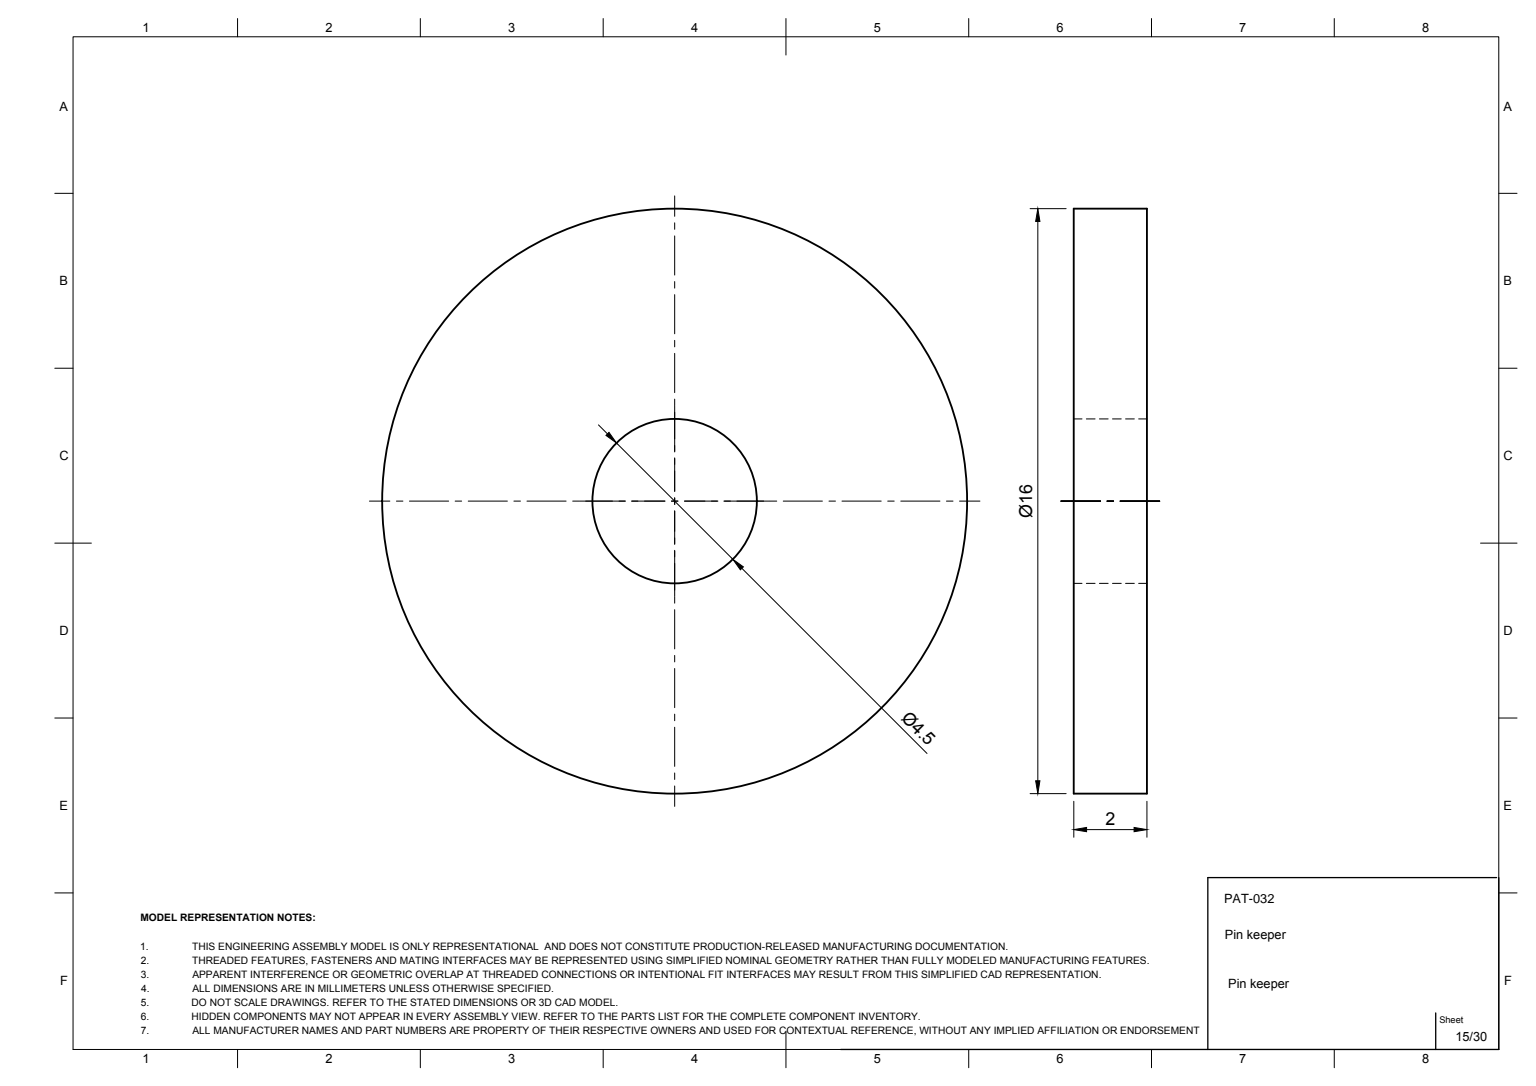
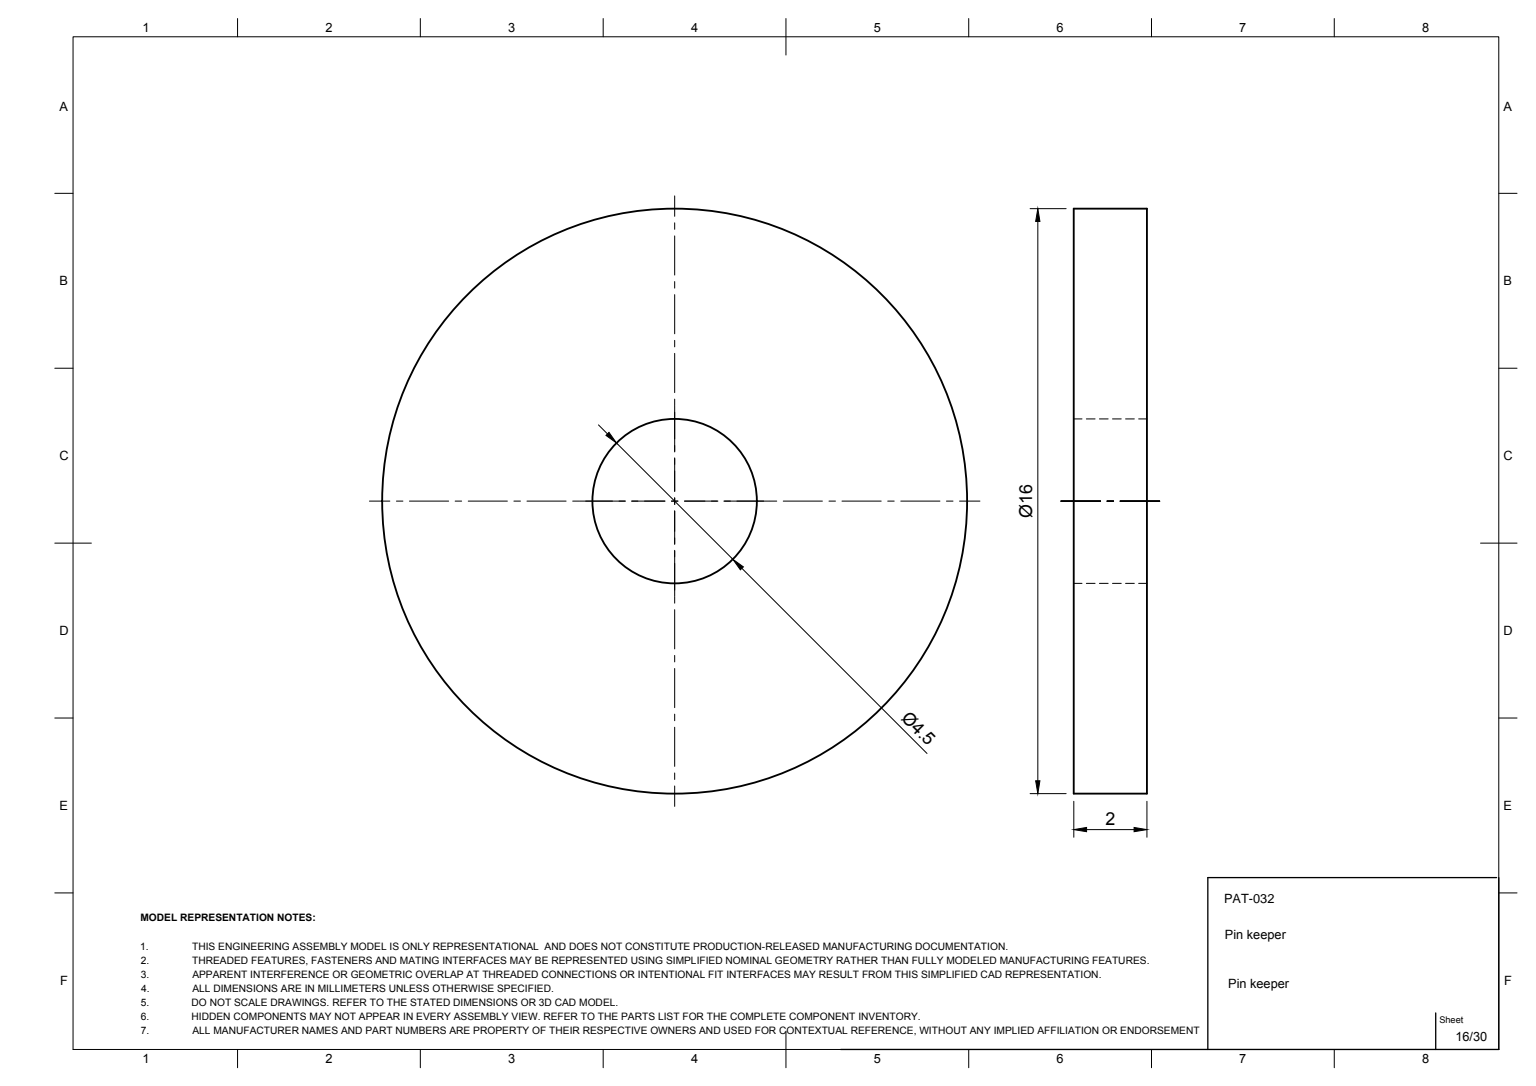
ISO-10303-21;
HEADER;
/* Generated by software containing ST-Developer
 * from STEP Tools, Inc. (www.steptools.com) 
 */

FILE_DESCRIPTION(
/* description */ ('Drill jig with bushing plate'),
/* implementation_level */ '2;1');

FILE_NAME(
/* name */ 'Pin keeper.step',
/* time_stamp */ '2026-10-27T10:51:08-07:00',
/* author */ (''),
/* organization */ (''),
/* preprocessor_version */ 'ST-DEVELOPER v20.2',
/* originating_system */ 'Autodesk Translation Framework v15.17.0.0',
/* authorisation */ '');

FILE_SCHEMA (('AUTOMOTIVE_DESIGN { 1 0 10303 214 3 1 1 }'));
ENDSEC;

DATA;
#10=MECHANICAL_DESIGN_GEOMETRIC_PRESENTATION_REPRESENTATION('',(#233),#6638);
#185=SHAPE_REPRESENTATION_RELATIONSHIP('SRR','None',#6749,#209);
#209=ADVANCED_BREP_SHAPE_REPRESENTATION('',(#257),#6622);
#233=STYLED_ITEM('',(#6943),#257);
#257=MANIFOLD_SOLID_BREP('Body1',#3600);
#330=FACE_BOUND('',#873,.T.);
#331=FACE_BOUND('',#875,.T.);
#427=PLANE('',#4068);
#428=PLANE('',#4069);
#595=FACE_OUTER_BOUND('',#870,.T.);
#596=FACE_OUTER_BOUND('',#871,.T.);
#597=FACE_OUTER_BOUND('',#872,.T.);
#598=FACE_OUTER_BOUND('',#874,.T.);
#870=EDGE_LOOP('',(#2831,#2832,#2833,#2834));
#871=EDGE_LOOP('',(#2835,#2836,#2837,#2838));
#872=EDGE_LOOP('',(#2839));
#873=EDGE_LOOP('',(#2840));
#874=EDGE_LOOP('',(#2841));
#875=EDGE_LOOP('',(#2842));
#1151=LINE('',#6024,#1412);
#1152=LINE('',#6030,#1413);
#1412=VECTOR('',#4816,0.225);
#1413=VECTOR('',#4823,0.8);
#1626=CIRCLE('',#4063,0.225);
#1627=CIRCLE('',#4064,0.225);
#1628=CIRCLE('',#4066,0.8);
#1629=CIRCLE('',#4067,0.8);
#1852=VERTEX_POINT('',#6021);
#1853=VERTEX_POINT('',#6023);
#1854=VERTEX_POINT('',#6027);
#1855=VERTEX_POINT('',#6029);
#2203=EDGE_CURVE('',#1852,#1852,#1626,.T.);
#2204=EDGE_CURVE('',#1852,#1853,#1151,.T.);
#2205=EDGE_CURVE('',#1853,#1853,#1627,.T.);
#2206=EDGE_CURVE('',#1854,#1854,#1628,.T.);
#2207=EDGE_CURVE('',#1854,#1855,#1152,.T.);
#2208=EDGE_CURVE('',#1855,#1855,#1629,.T.);
#2831=ORIENTED_EDGE('',*,*,#2203,.F.);
#2832=ORIENTED_EDGE('',*,*,#2204,.T.);
#2833=ORIENTED_EDGE('',*,*,#2205,.T.);
#2834=ORIENTED_EDGE('',*,*,#2204,.F.);
#2835=ORIENTED_EDGE('',*,*,#2206,.F.);
#2836=ORIENTED_EDGE('',*,*,#2207,.T.);
#2837=ORIENTED_EDGE('',*,*,#2208,.T.);
#2838=ORIENTED_EDGE('',*,*,#2207,.F.);
#2839=ORIENTED_EDGE('',*,*,#2206,.T.);
#2840=ORIENTED_EDGE('',*,*,#2203,.T.);
#2841=ORIENTED_EDGE('',*,*,#2208,.F.);
#2842=ORIENTED_EDGE('',*,*,#2205,.F.);
#3336=CYLINDRICAL_SURFACE('',#4062,0.225);
#3337=CYLINDRICAL_SURFACE('',#4065,0.8);
#3470=ADVANCED_FACE('',(#595),#3336,.F.);
#3471=ADVANCED_FACE('',(#596),#3337,.T.);
#3472=ADVANCED_FACE('',(#597,#330),#427,.T.);
#3473=ADVANCED_FACE('',(#598,#331),#428,.F.);
#3600=CLOSED_SHELL('',(#3470,#3471,#3472,#3473));
#4061=AXIS2_PLACEMENT_3D('',#6019,#4810,#4811);
#4062=AXIS2_PLACEMENT_3D('',#6020,#4812,#4813);
#4063=AXIS2_PLACEMENT_3D('',#6022,#4814,#4815);
#4064=AXIS2_PLACEMENT_3D('',#6025,#4817,#4818);
#4065=AXIS2_PLACEMENT_3D('',#6026,#4819,#4820);
#4066=AXIS2_PLACEMENT_3D('',#6028,#4821,#4822);
#4067=AXIS2_PLACEMENT_3D('',#6031,#4824,#4825);
#4068=AXIS2_PLACEMENT_3D('',#6032,#4826,#4827);
#4069=AXIS2_PLACEMENT_3D('',#6033,#4828,#4829);
#4810=DIRECTION('axis',(0.,0.,1.));
#4811=DIRECTION('refdir',(1.,0.,0.));
#4812=DIRECTION('center_axis',(1.,0.,0.));
#4813=DIRECTION('ref_axis',(0.,0.,-1.));
#4814=DIRECTION('center_axis',(-1.,0.,0.));
#4815=DIRECTION('ref_axis',(0.,0.,-1.));
#4816=DIRECTION('',(-1.,0.,0.));
#4817=DIRECTION('center_axis',(-1.,0.,0.));
#4818=DIRECTION('ref_axis',(0.,0.,-1.));
#4819=DIRECTION('center_axis',(1.,0.,0.));
#4820=DIRECTION('ref_axis',(0.,0.,-1.));
#4821=DIRECTION('center_axis',(1.,0.,0.));
#4822=DIRECTION('ref_axis',(0.,0.,-1.));
#4823=DIRECTION('',(-1.,0.,0.));
#4824=DIRECTION('center_axis',(1.,0.,0.));
#4825=DIRECTION('ref_axis',(0.,0.,-1.));
#4826=DIRECTION('center_axis',(1.,0.,0.));
#4827=DIRECTION('ref_axis',(0.,0.,-1.));
#4828=DIRECTION('center_axis',(1.,0.,0.));
#4829=DIRECTION('ref_axis',(0.,0.,-1.));
#6019=CARTESIAN_POINT('',(0.,0.,0.));
#6020=CARTESIAN_POINT('Origin',(-7.8,-6.,3.5));
#6021=CARTESIAN_POINT('',(-7.6,-6.,3.725));
#6022=CARTESIAN_POINT('Origin',(-7.6,-6.,3.5));
#6023=CARTESIAN_POINT('',(-7.8,-6.,3.725));
#6024=CARTESIAN_POINT('',(-7.8,-6.,3.725));
#6025=CARTESIAN_POINT('Origin',(-7.8,-6.,3.5));
#6026=CARTESIAN_POINT('Origin',(-7.8,-6.,3.5));
#6027=CARTESIAN_POINT('',(-7.6,-6.,4.3));
#6028=CARTESIAN_POINT('Origin',(-7.6,-6.,3.5));
#6029=CARTESIAN_POINT('',(-7.8,-6.,4.3));
#6030=CARTESIAN_POINT('',(-7.8,-6.,4.3));
#6031=CARTESIAN_POINT('Origin',(-7.8,-6.,3.5));
#6032=CARTESIAN_POINT('Origin',(-7.6,-6.,3.5));
#6033=CARTESIAN_POINT('Origin',(-7.8,-6.,3.5));
#6593=UNCERTAINTY_MEASURE_WITH_UNIT(LENGTH_MEASURE(0.001),#6639,
'DISTANCE_ACCURACY_VALUE',
'Maximum model space distance between geometric entities at asserted c
onnectivities');
#6609=UNCERTAINTY_MEASURE_WITH_UNIT(LENGTH_MEASURE(0.001),#6639,
'DISTANCE_ACCURACY_VALUE',
'Maximum model space distance between geometric entities at asserted c
onnectivities');
#6622=(
GEOMETRIC_REPRESENTATION_CONTEXT(3)
GLOBAL_UNCERTAINTY_ASSIGNED_CONTEXT((#6593))
GLOBAL_UNIT_ASSIGNED_CONTEXT((#6639,#6641,#6642))
REPRESENTATION_CONTEXT('','3D')
);
#6638=(
GEOMETRIC_REPRESENTATION_CONTEXT(3)
GLOBAL_UNCERTAINTY_ASSIGNED_CONTEXT((#6609))
GLOBAL_UNIT_ASSIGNED_CONTEXT((#6639,#6641,#6642))
REPRESENTATION_CONTEXT('','3D')
);
#6639=(
LENGTH_UNIT()
NAMED_UNIT(*)
SI_UNIT(.CENTI.,.METRE.)
);
#6641=(
NAMED_UNIT(*)
PLANE_ANGLE_UNIT()
SI_UNIT($,.RADIAN.)
);
#6642=(
NAMED_UNIT(*)
SI_UNIT($,.STERADIAN.)
SOLID_ANGLE_UNIT()
);
#6655=SHAPE_DEFINITION_REPRESENTATION(#6683,#6749);
#6683=PRODUCT_DEFINITION_SHAPE('',$,#6778);
#6749=SHAPE_REPRESENTATION('',(#4061),#6622);
#6765=PRODUCT_DEFINITION_CONTEXT('part definition',#6851,'design');
#6778=PRODUCT_DEFINITION('Pin keeper','Pin keeper',#6806,#6765);
#6806=PRODUCT_DEFINITION_FORMATION('',$,#6865);
#6851=APPLICATION_CONTEXT(
'Core Data for Automotive Mechanical Design Process');
#6852=PRODUCT_CONTEXT('part definition',#6851,'mechanical');
#6865=PRODUCT('Pin keeper','Pin keeper','Pin keeper',(#6852));
#6937=COLOUR_RGB('Grey',0.48,0.52,0.57);
#6938=FILL_AREA_STYLE_COLOUR('',#6937);
#6939=FILL_AREA_STYLE('',(#6938));
#6940=SURFACE_STYLE_FILL_AREA(#6939);
#6941=SURFACE_SIDE_STYLE('',(#6940));
#6942=SURFACE_STYLE_USAGE(.BOTH.,#6941);
#6943=PRESENTATION_STYLE_ASSIGNMENT((#6942));
ENDSEC;
END-ISO-10303-21;
